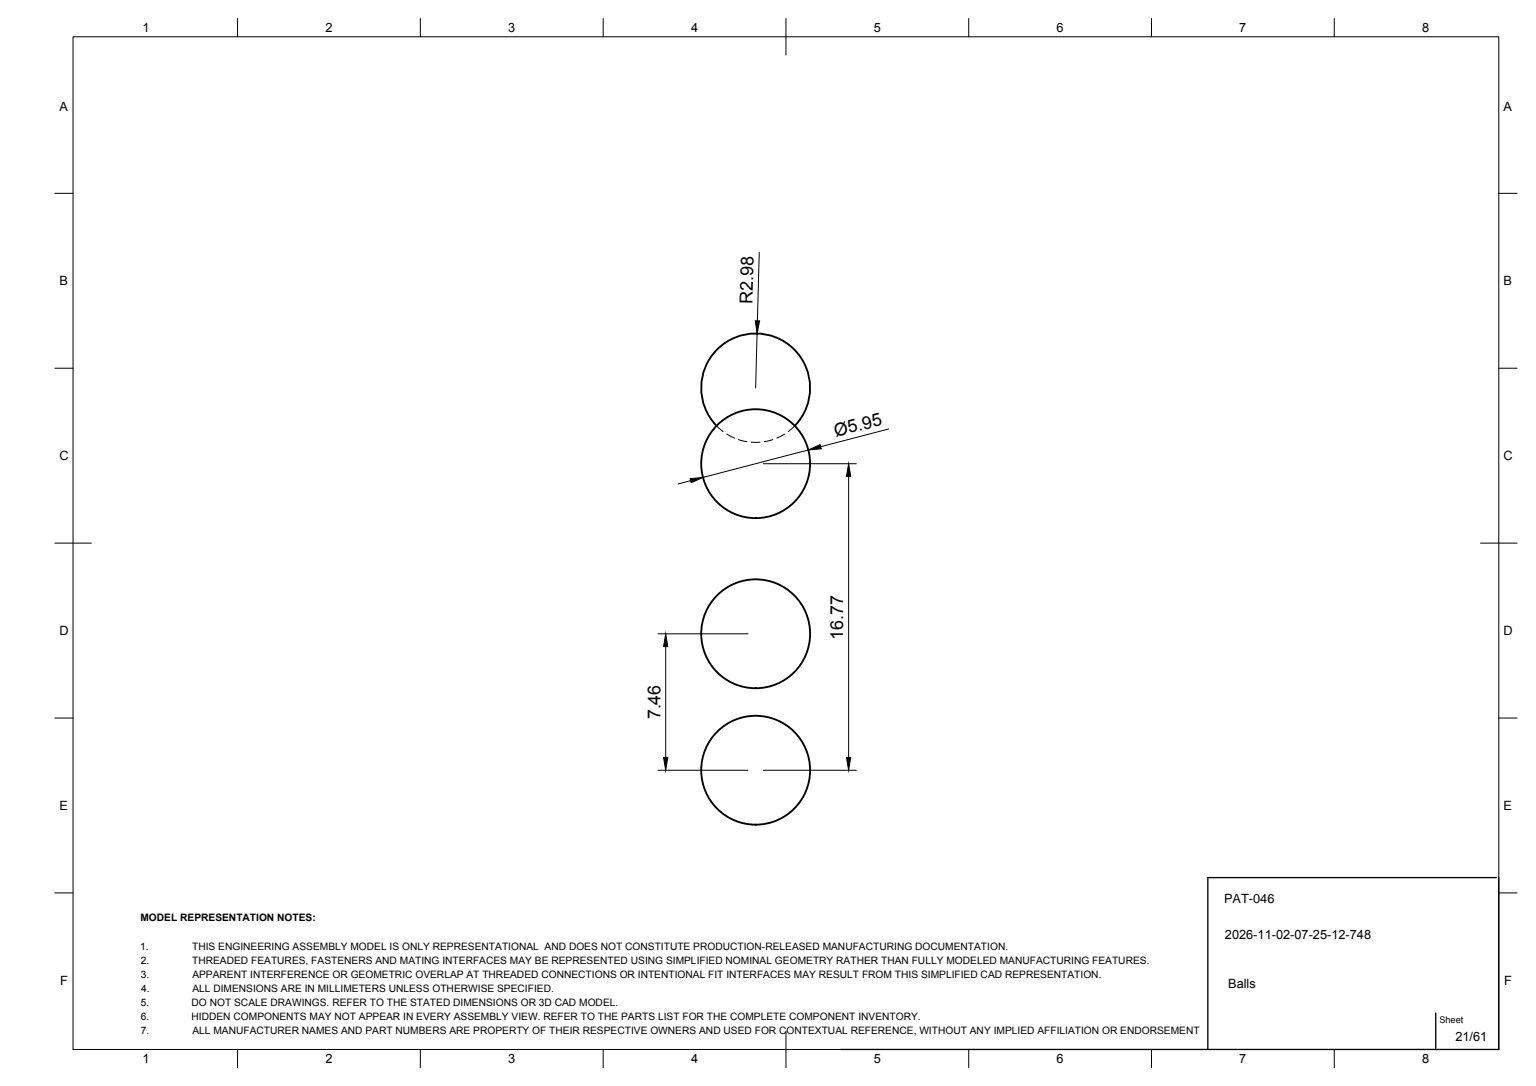
ISO-10303-21;
HEADER;
/* Generated by software containing ST-Developer
 * from STEP Tools, Inc. (www.steptools.com) 
 */

FILE_DESCRIPTION(
/* description */ ('Gear mesh backlash fixture'),
/* implementation_level */ '2;1');

FILE_NAME(
/* name */ 'Balls.step',
/* time_stamp */ '2026-10-28T03:26:00-07:00',
/* author */ (''),
/* organization */ (''),
/* preprocessor_version */ 'ST-DEVELOPER v20.2',
/* originating_system */ 'Autodesk Translation Framework v15.17.0.0',
/* authorisation */ '');

FILE_SCHEMA (('AUTOMOTIVE_DESIGN { 1 0 10303 214 3 1 1 }'));
ENDSEC;

DATA;
#10=MECHANICAL_DESIGN_GEOMETRIC_PRESENTATION_REPRESENTATION('',(#1030,#1031,#1032,#1033,#1034,#1035,#1036),#57900);
#729=SPHERICAL_SURFACE('',#14538,0.29765);
#730=SPHERICAL_SURFACE('',#14540,0.29765);
#731=SPHERICAL_SURFACE('',#14542,0.29765);
#732=SPHERICAL_SURFACE('',#14544,0.29765);
#733=SPHERICAL_SURFACE('',#14546,0.29765);
#734=SPHERICAL_SURFACE('',#14548,0.29765);
#735=SPHERICAL_SURFACE('',#14550,0.29765);
#930=SHAPE_REPRESENTATION_RELATIONSHIP('SRR','None',#58126,#980);
#980=ADVANCED_BREP_SHAPE_REPRESENTATION('',(#1095,#1096,#1097,#1098,#1099,
#1100,#1101),#57859);
#1030=STYLED_ITEM('',(#58465),#1095);
#1031=STYLED_ITEM('',(#58465),#1096);
#1032=STYLED_ITEM('',(#58465),#1097);
#1033=STYLED_ITEM('',(#58465),#1098);
#1034=STYLED_ITEM('',(#58465),#1099);
#1035=STYLED_ITEM('',(#58465),#1100);
#1036=STYLED_ITEM('',(#58465),#1101);
#1095=MANIFOLD_SOLID_BREP('Body1',#13590);
#1096=MANIFOLD_SOLID_BREP('Body2',#13591);
#1097=MANIFOLD_SOLID_BREP('Body3',#13592);
#1098=MANIFOLD_SOLID_BREP('Body4',#13593);
#1099=MANIFOLD_SOLID_BREP('Body5',#13594);
#1100=MANIFOLD_SOLID_BREP('Body6',#13595);
#1101=MANIFOLD_SOLID_BREP('Body7',#13596);
#1856=FACE_OUTER_BOUND('',#2699,.T.);
#1857=FACE_OUTER_BOUND('',#2700,.T.);
#1858=FACE_OUTER_BOUND('',#2701,.T.);
#1859=FACE_OUTER_BOUND('',#2702,.T.);
#1860=FACE_OUTER_BOUND('',#2703,.T.);
#1861=FACE_OUTER_BOUND('',#2704,.T.);
#1862=FACE_OUTER_BOUND('',#2705,.T.);
#2699=EDGE_LOOP('',(#9611,#9612));
#2700=EDGE_LOOP('',(#9613,#9614));
#2701=EDGE_LOOP('',(#9615,#9616));
#2702=EDGE_LOOP('',(#9617,#9618));
#2703=EDGE_LOOP('',(#9619,#9620));
#2704=EDGE_LOOP('',(#9621,#9622));
#2705=EDGE_LOOP('',(#9623,#9624));
#5352=CIRCLE('',#14539,0.29765);
#5353=CIRCLE('',#14541,0.29765);
#5354=CIRCLE('',#14543,0.29765);
#5355=CIRCLE('',#14545,0.29765);
#5356=CIRCLE('',#14547,0.29765);
#5357=CIRCLE('',#14549,0.29765);
#5358=CIRCLE('',#14551,0.29765);
#6019=VERTEX_POINT('',#20113);
#6020=VERTEX_POINT('',#20114);
#6021=VERTEX_POINT('',#20117);
#6022=VERTEX_POINT('',#20118);
#6023=VERTEX_POINT('',#20121);
#6024=VERTEX_POINT('',#20122);
#6025=VERTEX_POINT('',#20125);
#6026=VERTEX_POINT('',#20126);
#6027=VERTEX_POINT('',#20129);
#6028=VERTEX_POINT('',#20130);
#6029=VERTEX_POINT('',#20133);
#6030=VERTEX_POINT('',#20134);
#6031=VERTEX_POINT('',#20137);
#6032=VERTEX_POINT('',#20138);
#7392=EDGE_CURVE('',#6019,#6020,#5352,.T.);
#7393=EDGE_CURVE('',#6021,#6022,#5353,.T.);
#7394=EDGE_CURVE('',#6023,#6024,#5354,.T.);
#7395=EDGE_CURVE('',#6025,#6026,#5355,.T.);
#7396=EDGE_CURVE('',#6027,#6028,#5356,.T.);
#7397=EDGE_CURVE('',#6029,#6030,#5357,.T.);
#7398=EDGE_CURVE('',#6031,#6032,#5358,.T.);
#9611=ORIENTED_EDGE('',*,*,#7392,.T.);
#9612=ORIENTED_EDGE('',*,*,#7392,.F.);
#9613=ORIENTED_EDGE('',*,*,#7393,.T.);
#9614=ORIENTED_EDGE('',*,*,#7393,.F.);
#9615=ORIENTED_EDGE('',*,*,#7394,.T.);
#9616=ORIENTED_EDGE('',*,*,#7394,.F.);
#9617=ORIENTED_EDGE('',*,*,#7395,.T.);
#9618=ORIENTED_EDGE('',*,*,#7395,.F.);
#9619=ORIENTED_EDGE('',*,*,#7396,.T.);
#9620=ORIENTED_EDGE('',*,*,#7396,.F.);
#9621=ORIENTED_EDGE('',*,*,#7397,.T.);
#9622=ORIENTED_EDGE('',*,*,#7397,.F.);
#9623=ORIENTED_EDGE('',*,*,#7398,.T.);
#9624=ORIENTED_EDGE('',*,*,#7398,.F.);
#12973=ADVANCED_FACE('',(#1856),#729,.T.);
#12974=ADVANCED_FACE('',(#1857),#730,.T.);
#12975=ADVANCED_FACE('',(#1858),#731,.T.);
#12976=ADVANCED_FACE('',(#1859),#732,.T.);
#12977=ADVANCED_FACE('',(#1860),#733,.T.);
#12978=ADVANCED_FACE('',(#1861),#734,.T.);
#12979=ADVANCED_FACE('',(#1862),#735,.T.);
#13590=CLOSED_SHELL('',(#12973));
#13591=CLOSED_SHELL('',(#12974));
#13592=CLOSED_SHELL('',(#12975));
#13593=CLOSED_SHELL('',(#12976));
#13594=CLOSED_SHELL('',(#12977));
#13595=CLOSED_SHELL('',(#12978));
#13596=CLOSED_SHELL('',(#12979));
#14537=AXIS2_PLACEMENT_3D('',#20111,#16458,#16459);
#14538=AXIS2_PLACEMENT_3D('',#20112,#16460,#16461);
#14539=AXIS2_PLACEMENT_3D('',#20115,#16462,#16463);
#14540=AXIS2_PLACEMENT_3D('',#20116,#16464,#16465);
#14541=AXIS2_PLACEMENT_3D('',#20119,#16466,#16467);
#14542=AXIS2_PLACEMENT_3D('',#20120,#16468,#16469);
#14543=AXIS2_PLACEMENT_3D('',#20123,#16470,#16471);
#14544=AXIS2_PLACEMENT_3D('',#20124,#16472,#16473);
#14545=AXIS2_PLACEMENT_3D('',#20127,#16474,#16475);
#14546=AXIS2_PLACEMENT_3D('',#20128,#16476,#16477);
#14547=AXIS2_PLACEMENT_3D('',#20131,#16478,#16479);
#14548=AXIS2_PLACEMENT_3D('',#20132,#16480,#16481);
#14549=AXIS2_PLACEMENT_3D('',#20135,#16482,#16483);
#14550=AXIS2_PLACEMENT_3D('',#20136,#16484,#16485);
#14551=AXIS2_PLACEMENT_3D('',#20139,#16486,#16487);
#16458=DIRECTION('axis',(0.,0.,1.));
#16459=DIRECTION('refdir',(1.,0.,0.));
#16460=DIRECTION('center_axis',(0.,0.,1.));
#16461=DIRECTION('ref_axis',(1.,0.,0.));
#16462=DIRECTION('center_axis',(1.22464679914735E-16,-1.,0.));
#16463=DIRECTION('ref_axis',(-1.,-1.22464679914735E-16,0.));
#16464=DIRECTION('center_axis',(0.78183148246803,0.,0.623489801858733));
#16465=DIRECTION('ref_axis',(0.623489801858734,0.,-0.78183148246803));
#16466=DIRECTION('center_axis',(7.63554790147315E-17,-1.,-9.57467422477103E-17));
#16467=DIRECTION('ref_axis',(-0.623489801858734,-1.22464679914735E-16,0.78183148246803));
#16468=DIRECTION('center_axis',(0.974927912181824,0.,-0.222520933956314));
#16469=DIRECTION('ref_axis',(-0.222520933956314,0.,-0.974927912181824));
#16470=DIRECTION('center_axis',(-2.7250954951288E-17,-1.,-1.19394234705288E-16));
#16471=DIRECTION('ref_axis',(0.222520933956314,-1.22464679914735E-16,0.974927912181824));
#16472=DIRECTION('center_axis',(0.433883739117558,0.,-0.900968867902419));
#16473=DIRECTION('ref_axis',(-0.900968867902419,0.,-0.433883739117558));
#16474=DIRECTION('center_axis',(-1.10336864020811E-16,-1.,-5.31354332312403E-17));
#16475=DIRECTION('ref_axis',(0.900968867902419,-1.22464679914735E-16,0.433883739117558));
#16476=DIRECTION('center_axis',(-0.433883739117558,0.,-0.900968867902419));
#16477=DIRECTION('ref_axis',(-0.900968867902419,0.,0.433883739117558));
#16478=DIRECTION('center_axis',(-1.10336864020811E-16,-1.,5.31354332312403E-17));
#16479=DIRECTION('ref_axis',(0.900968867902419,-1.22464679914735E-16,-0.433883739117558));
#16480=DIRECTION('center_axis',(-0.974927912181824,0.,-0.222520933956314));
#16481=DIRECTION('ref_axis',(-0.222520933956315,0.,0.974927912181824));
#16482=DIRECTION('center_axis',(-2.7250954951288E-17,-1.,1.19394234705288E-16));
#16483=DIRECTION('ref_axis',(0.222520933956315,-1.22464679914735E-16,-0.974927912181824));
#16484=DIRECTION('center_axis',(-0.78183148246803,0.,0.623489801858734));
#16485=DIRECTION('ref_axis',(0.623489801858733,0.,0.78183148246803));
#16486=DIRECTION('center_axis',(7.63554790147315E-17,-1.,9.57467422477103E-17));
#16487=DIRECTION('ref_axis',(-0.623489801858733,-1.22464679914735E-16,-0.78183148246803));
#20111=CARTESIAN_POINT('',(0.,0.,0.));
#20112=CARTESIAN_POINT('Origin',(1.1,0.,0.));
#20113=CARTESIAN_POINT('',(1.1,-2.23201749654651E-33,0.29765));
#20114=CARTESIAN_POINT('',(1.1,-2.23201749654651E-33,-0.29765));
#20115=CARTESIAN_POINT('Origin',(1.1,0.,0.));
#20116=CARTESIAN_POINT('Origin',(0.685838782044607,0.,-0.860014630714833));
#20117=CARTESIAN_POINT('',(0.918550922801216,-5.31350540756609E-33,-0.674432891191581));
#20118=CARTESIAN_POINT('',(0.453126641287998,8.49470414473068E-34,-1.04559637023808));
#20119=CARTESIAN_POINT('Origin',(0.685838782044607,0.,-0.860014630714833));
#20120=CARTESIAN_POINT('Origin',(-0.244773027351946,0.,-1.07242070340001));
#20121=CARTESIAN_POINT('',(0.0454142657089739,-2.23201749654651E-33,-1.1386540593921));
#20122=CARTESIAN_POINT('',(-0.534960320412865,-2.23201749654651E-33,-1.00618734740791));
#20123=CARTESIAN_POINT('Origin',(-0.244773027351946,0.,-1.07242070340001));
#20124=CARTESIAN_POINT('Origin',(-0.991065754692661,0.,-0.477272113029314));
#20125=CARTESIAN_POINT('',(-0.86192025974432,8.49470414473067E-34,-0.745445496560469));
#20126=CARTESIAN_POINT('',(-1.120211249641,-5.31350540756609E-33,-0.209098729498159));
#20127=CARTESIAN_POINT('Origin',(-0.991065754692661,0.,-0.477272113029314));
#20128=CARTESIAN_POINT('Origin',(-0.991065754692661,0.,0.477272113029314));
#20129=CARTESIAN_POINT('',(-1.120211249641,-2.23201749654651E-33,0.209098729498159));
#20130=CARTESIAN_POINT('',(-0.86192025974432,-2.23201749654651E-33,0.745445496560469));
#20131=CARTESIAN_POINT('Origin',(-0.991065754692661,0.,0.477272113029314));
#20132=CARTESIAN_POINT('Origin',(-0.244773027351946,0.,1.07242070340001));
#20133=CARTESIAN_POINT('',(-0.534960320412866,-2.23201749654651E-33,1.00618734740791));
#20134=CARTESIAN_POINT('',(0.0454142657089737,-2.23201749654651E-33,1.1386540593921));
#20135=CARTESIAN_POINT('Origin',(-0.244773027351946,0.,1.07242070340001));
#20136=CARTESIAN_POINT('Origin',(0.685838782044607,0.,0.860014630714833));
#20137=CARTESIAN_POINT('',(0.453126641287998,-2.23201749654651E-33,1.04559637023808));
#20138=CARTESIAN_POINT('',(0.918550922801216,-2.23201749654651E-33,0.674432891191581));
#20139=CARTESIAN_POINT('Origin',(0.685838782044607,0.,0.860014630714833));
#57800=UNCERTAINTY_MEASURE_WITH_UNIT(LENGTH_MEASURE(0.001),#57901,
'DISTANCE_ACCURACY_VALUE',
'Maximum model space distance between geometric entities at asserted c
onnectivities');
#57841=UNCERTAINTY_MEASURE_WITH_UNIT(LENGTH_MEASURE(0.001),#57901,
'DISTANCE_ACCURACY_VALUE',
'Maximum model space distance between geometric entities at asserted c
onnectivities');
#57859=(
GEOMETRIC_REPRESENTATION_CONTEXT(3)
GLOBAL_UNCERTAINTY_ASSIGNED_CONTEXT((#57800))
GLOBAL_UNIT_ASSIGNED_CONTEXT((#57901,#57903,#57904))
REPRESENTATION_CONTEXT('','3D')
);
#57900=(
GEOMETRIC_REPRESENTATION_CONTEXT(3)
GLOBAL_UNCERTAINTY_ASSIGNED_CONTEXT((#57841))
GLOBAL_UNIT_ASSIGNED_CONTEXT((#57901,#57903,#57904))
REPRESENTATION_CONTEXT('','3D')
);
#57901=(
LENGTH_UNIT()
NAMED_UNIT(*)
SI_UNIT(.CENTI.,.METRE.)
);
#57903=(
NAMED_UNIT(*)
PLANE_ANGLE_UNIT()
SI_UNIT($,.RADIAN.)
);
#57904=(
NAMED_UNIT(*)
SI_UNIT($,.STERADIAN.)
SOLID_ANGLE_UNIT()
);
#57922=SHAPE_DEFINITION_REPRESENTATION(#57980,#58126);
#57980=PRODUCT_DEFINITION_SHAPE('',$,#58185);
#58126=SHAPE_REPRESENTATION('',(#14537),#57859);
#58167=PRODUCT_DEFINITION_CONTEXT('part definition',#58343,'design');
#58185=PRODUCT_DEFINITION('Balls','Balls',#58243,#58167);
#58243=PRODUCT_DEFINITION_FORMATION('',$,#58362);
#58343=APPLICATION_CONTEXT(
'Core Data for Automotive Mechanical Design Process');
#58344=PRODUCT_CONTEXT('part definition',#58343,'mechanical');
#58362=PRODUCT('Balls','Balls','Balls',(#58344));
#58459=COLOUR_RGB('Grey',0.48,0.52,0.57);
#58460=FILL_AREA_STYLE_COLOUR('',#58459);
#58461=FILL_AREA_STYLE('',(#58460));
#58462=SURFACE_STYLE_FILL_AREA(#58461);
#58463=SURFACE_SIDE_STYLE('',(#58462));
#58464=SURFACE_STYLE_USAGE(.BOTH.,#58463);
#58465=PRESENTATION_STYLE_ASSIGNMENT((#58464));
ENDSEC;
END-ISO-10303-21;
